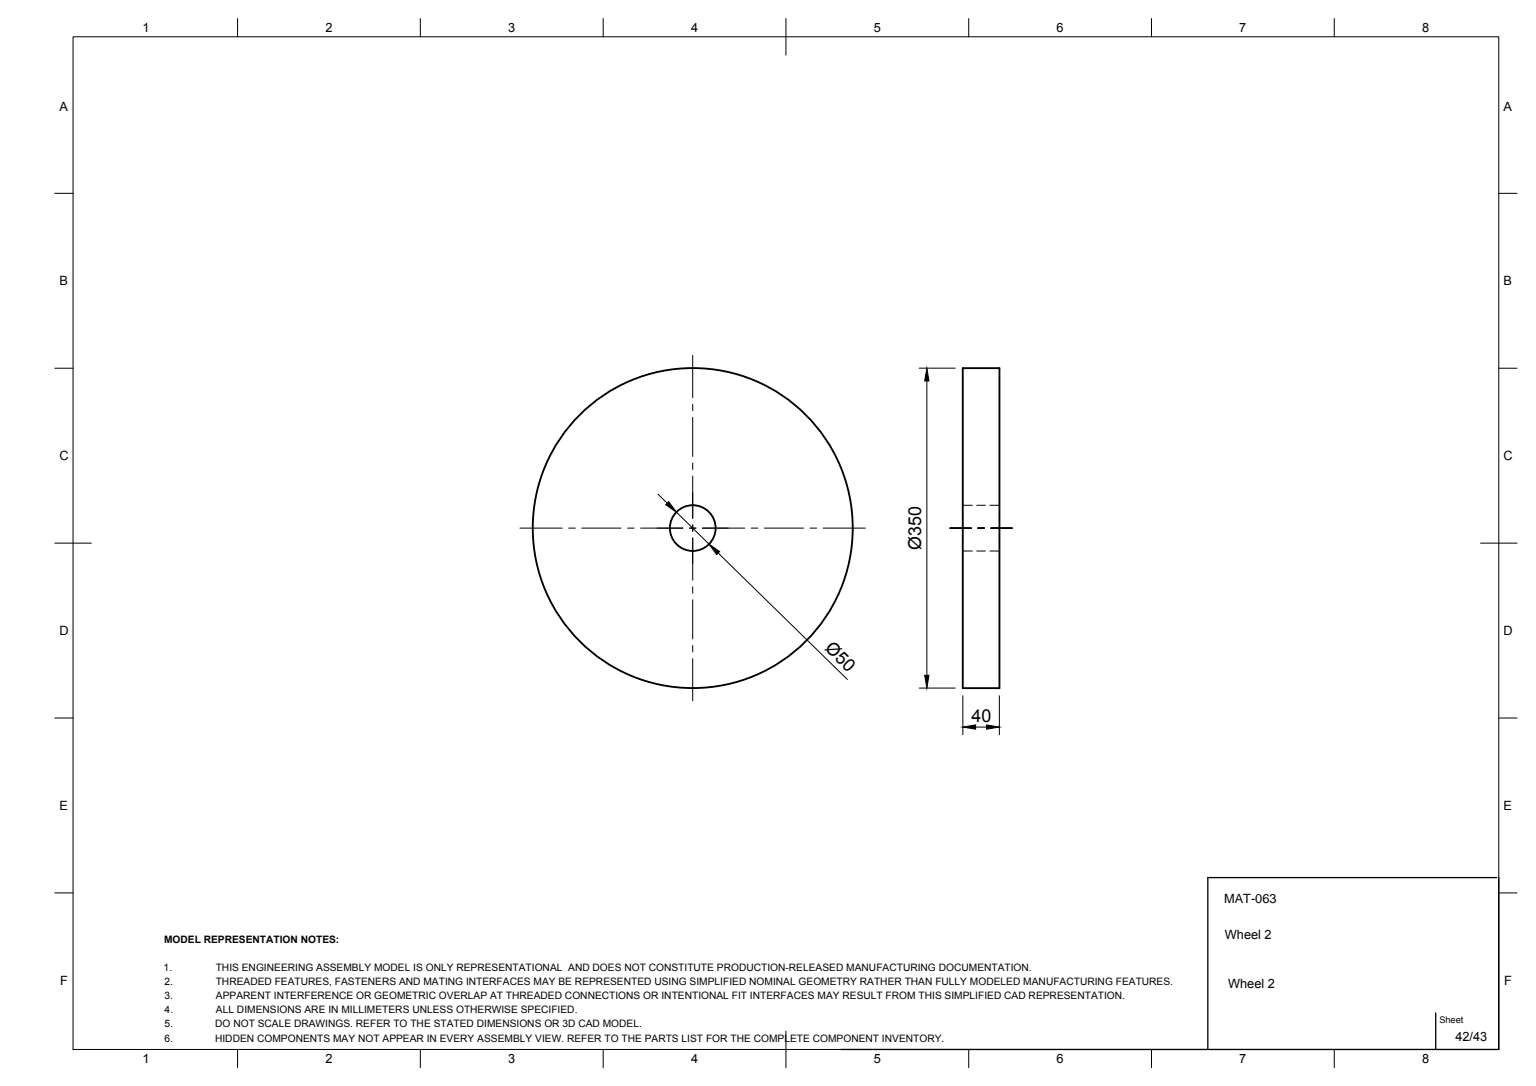
ISO-10303-21;
HEADER;
/* Generated by software containing ST-Developer
 * from STEP Tools, Inc. (www.steptools.com) 
 */

FILE_DESCRIPTION(
/* description */ (''),
/* implementation_level */ '2;1');

FILE_NAME(
/* name */ 'Wheel 2.step',
/* time_stamp */ '2026-10-24T09:43:01-07:00',
/* author */ (''),
/* organization */ (''),
/* preprocessor_version */ 'ST-DEVELOPER v20.2',
/* originating_system */ 'Autodesk Translation Framework v15.15.0.0',
/* authorisation */ '');

FILE_SCHEMA (('AUTOMOTIVE_DESIGN { 1 0 10303 214 3 1 1 }'));
ENDSEC;

DATA;
#10=MECHANICAL_DESIGN_GEOMETRIC_PRESENTATION_REPRESENTATION('',(#304),#11112);
#238=SHAPE_REPRESENTATION_RELATIONSHIP('SRR','None',#11265,#271);
#271=ADVANCED_BREP_SHAPE_REPRESENTATION('',(#337),#11110);
#304=STYLED_ITEM('',(#11426),#337);
#337=MANIFOLD_SOLID_BREP('Wheel 2',#6041);
#494=FACE_BOUND('',#1551,.T.);
#495=FACE_BOUND('',#1553,.T.);
#661=PLANE('',#7230);
#662=PLANE('',#7232);
#1030=FACE_OUTER_BOUND('',#1549,.T.);
#1031=FACE_OUTER_BOUND('',#1550,.T.);
#1032=FACE_OUTER_BOUND('',#1552,.T.);
#1033=FACE_OUTER_BOUND('',#1554,.T.);
#1549=EDGE_LOOP('',(#5481,#5482,#5483,#5484));
#1550=EDGE_LOOP('',(#5485));
#1551=EDGE_LOOP('',(#5486));
#1552=EDGE_LOOP('',(#5487));
#1553=EDGE_LOOP('',(#5488));
#1554=EDGE_LOOP('',(#5489,#5490,#5491,#5492));
#1914=LINE('',#10997,#2273);
#1915=LINE('',#11006,#2274);
#2273=VECTOR('',#9260,0.025);
#2274=VECTOR('',#9273,0.174999999);
#2676=CIRCLE('',#7228,0.025);
#2677=CIRCLE('',#7229,0.025);
#2678=CIRCLE('',#7231,0.174999999);
#2679=CIRCLE('',#7233,0.174999999);
#3174=VERTEX_POINT('',#10994);
#3175=VERTEX_POINT('',#10996);
#3176=VERTEX_POINT('',#11000);
#3177=VERTEX_POINT('',#11003);
#3944=EDGE_CURVE('',#3174,#3174,#2676,.T.);
#3945=EDGE_CURVE('',#3174,#3175,#1914,.T.);
#3946=EDGE_CURVE('',#3175,#3175,#2677,.F.);
#3947=EDGE_CURVE('',#3176,#3176,#2678,.F.);
#3948=EDGE_CURVE('',#3177,#3177,#2679,.F.);
#3949=EDGE_CURVE('',#3176,#3177,#1915,.T.);
#5481=ORIENTED_EDGE('',*,*,#3944,.F.);
#5482=ORIENTED_EDGE('',*,*,#3945,.T.);
#5483=ORIENTED_EDGE('',*,*,#3946,.F.);
#5484=ORIENTED_EDGE('',*,*,#3945,.F.);
#5485=ORIENTED_EDGE('',*,*,#3947,.F.);
#5486=ORIENTED_EDGE('',*,*,#3946,.T.);
#5487=ORIENTED_EDGE('',*,*,#3948,.T.);
#5488=ORIENTED_EDGE('',*,*,#3944,.T.);
#5489=ORIENTED_EDGE('',*,*,#3947,.T.);
#5490=ORIENTED_EDGE('',*,*,#3949,.T.);
#5491=ORIENTED_EDGE('',*,*,#3948,.F.);
#5492=ORIENTED_EDGE('',*,*,#3949,.F.);
#5643=CYLINDRICAL_SURFACE('',#7227,0.025);
#5644=CYLINDRICAL_SURFACE('',#7234,0.174999999);
#6003=ADVANCED_FACE('',(#1030),#5643,.F.);
#6004=ADVANCED_FACE('',(#1031,#494),#661,.F.);
#6005=ADVANCED_FACE('',(#1032,#495),#662,.T.);
#6006=ADVANCED_FACE('',(#1033),#5644,.T.);
#6041=CLOSED_SHELL('',(#6003,#6004,#6005,#6006));
#7226=AXIS2_PLACEMENT_3D('',#10992,#9254,#9255);
#7227=AXIS2_PLACEMENT_3D('',#10993,#9256,#9257);
#7228=AXIS2_PLACEMENT_3D('',#10995,#9258,#9259);
#7229=AXIS2_PLACEMENT_3D('',#10998,#9261,#9262);
#7230=AXIS2_PLACEMENT_3D('',#10999,#9263,#9264);
#7231=AXIS2_PLACEMENT_3D('',#11001,#9265,#9266);
#7232=AXIS2_PLACEMENT_3D('',#11002,#9267,#9268);
#7233=AXIS2_PLACEMENT_3D('',#11004,#9269,#9270);
#7234=AXIS2_PLACEMENT_3D('',#11005,#9271,#9272);
#9254=DIRECTION('axis',(0.,0.,1.));
#9255=DIRECTION('refdir',(1.,0.,0.));
#9256=DIRECTION('center_axis',(1.,0.,0.));
#9257=DIRECTION('ref_axis',(0.,0.,-1.));
#9258=DIRECTION('center_axis',(1.,0.,0.));
#9259=DIRECTION('ref_axis',(0.,0.,-1.));
#9260=DIRECTION('',(1.,0.,0.));
#9261=DIRECTION('center_axis',(1.,0.,0.));
#9262=DIRECTION('ref_axis',(0.,0.,-1.));
#9263=DIRECTION('center_axis',(-1.,-4.89404439732087E-17,-4.89404438350122E-17));
#9264=DIRECTION('ref_axis',(4.89404439732087E-17,-1.,5.74495806648814E-50));
#9265=DIRECTION('center_axis',(1.,0.,0.));
#9266=DIRECTION('ref_axis',(0.,0.,-1.));
#9267=DIRECTION('center_axis',(-1.,0.,0.));
#9268=DIRECTION('ref_axis',(0.,0.,1.));
#9269=DIRECTION('center_axis',(1.,0.,0.));
#9270=DIRECTION('ref_axis',(0.,0.,-1.));
#9271=DIRECTION('center_axis',(1.,0.,0.));
#9272=DIRECTION('ref_axis',(0.,0.,-1.));
#9273=DIRECTION('',(-1.,0.,0.));
#10992=CARTESIAN_POINT('',(0.,0.,0.));
#10993=CARTESIAN_POINT('Origin',(-0.595,-0.386547301,0.));
#10994=CARTESIAN_POINT('',(-0.595,-0.386547301,0.025));
#10995=CARTESIAN_POINT('Origin',(-0.595,-0.386547301,0.));
#10996=CARTESIAN_POINT('',(-0.555,-0.386547301,0.025));
#10997=CARTESIAN_POINT('',(-0.595,-0.386547301,0.025));
#10998=CARTESIAN_POINT('Origin',(-0.555,-0.386547301,0.));
#10999=CARTESIAN_POINT('Origin',(-0.555,-0.3865473015,4.16333634234433E-19));
#11000=CARTESIAN_POINT('',(-0.555,-0.386547301,0.174999999));
#11001=CARTESIAN_POINT('Origin',(-0.555,-0.386547301,0.));
#11002=CARTESIAN_POINT('Origin',(-0.595,-0.3865473015,4.16333634234433E-19));
#11003=CARTESIAN_POINT('',(-0.595,-0.386547301,0.174999999));
#11004=CARTESIAN_POINT('Origin',(-0.595,-0.386547301,0.));
#11005=CARTESIAN_POINT('Origin',(-0.595,-0.386547301,0.));
#11006=CARTESIAN_POINT('',(-0.595,-0.386547301,0.174999999));
#11071=UNCERTAINTY_MEASURE_WITH_UNIT(LENGTH_MEASURE(1.E-5),#11113,
'DISTANCE_ACCURACY_VALUE',
'Maximum model space distance between geometric entities at asserted c
onnectivities');
#11073=UNCERTAINTY_MEASURE_WITH_UNIT(LENGTH_MEASURE(1.E-5),#11113,
'DISTANCE_ACCURACY_VALUE',
'Maximum model space distance between geometric entities at asserted c
onnectivities');
#11110=(
GEOMETRIC_REPRESENTATION_CONTEXT(3)
GLOBAL_UNCERTAINTY_ASSIGNED_CONTEXT((#11071))
GLOBAL_UNIT_ASSIGNED_CONTEXT((#11113,#11114,#11115))
REPRESENTATION_CONTEXT('','3D')
);
#11112=(
GEOMETRIC_REPRESENTATION_CONTEXT(3)
GLOBAL_UNCERTAINTY_ASSIGNED_CONTEXT((#11073))
GLOBAL_UNIT_ASSIGNED_CONTEXT((#11113,#11114,#11115))
REPRESENTATION_CONTEXT('','3D')
);
#11113=(
LENGTH_UNIT()
NAMED_UNIT(*)
SI_UNIT($,.METRE.)
);
#11114=(
NAMED_UNIT(*)
PLANE_ANGLE_UNIT()
SI_UNIT($,.RADIAN.)
);
#11115=(
NAMED_UNIT(*)
SI_UNIT($,.STERADIAN.)
SOLID_ANGLE_UNIT()
);
#11152=SHAPE_DEFINITION_REPRESENTATION(#11208,#11265);
#11208=PRODUCT_DEFINITION_SHAPE('',$,#11304);
#11265=SHAPE_REPRESENTATION('',(#7226),#11110);
#11267=PRODUCT_DEFINITION_CONTEXT('part definition',#11383,'design');
#11304=PRODUCT_DEFINITION('Wheel 2','Wheel 2',#11342,#11267);
#11342=PRODUCT_DEFINITION_FORMATION('',$,#11421);
#11383=APPLICATION_CONTEXT(
'Core Data for Automotive Mechanical Design Process');
#11384=PRODUCT_CONTEXT('part definition',#11383,'mechanical');
#11421=PRODUCT('Wheel 2','Wheel 2','wheel__ DE     9613',(#11384));
#11426=PRESENTATION_STYLE_ASSIGNMENT((#11430));
#11430=SURFACE_STYLE_USAGE(.BOTH.,#11434);
#11434=SURFACE_SIDE_STYLE('',(#11438));
#11438=SURFACE_STYLE_FILL_AREA(#11442);
#11442=FILL_AREA_STYLE('Opaque(202,209,238)',(#11446));
#11446=FILL_AREA_STYLE_COLOUR('Opaque(202,209,238)',#11450);
#11450=COLOUR_RGB('Opaque(202,209,238)',0.792156862745098,0.819607843137255,
0.933333333333333);
ENDSEC;
END-ISO-10303-21;
